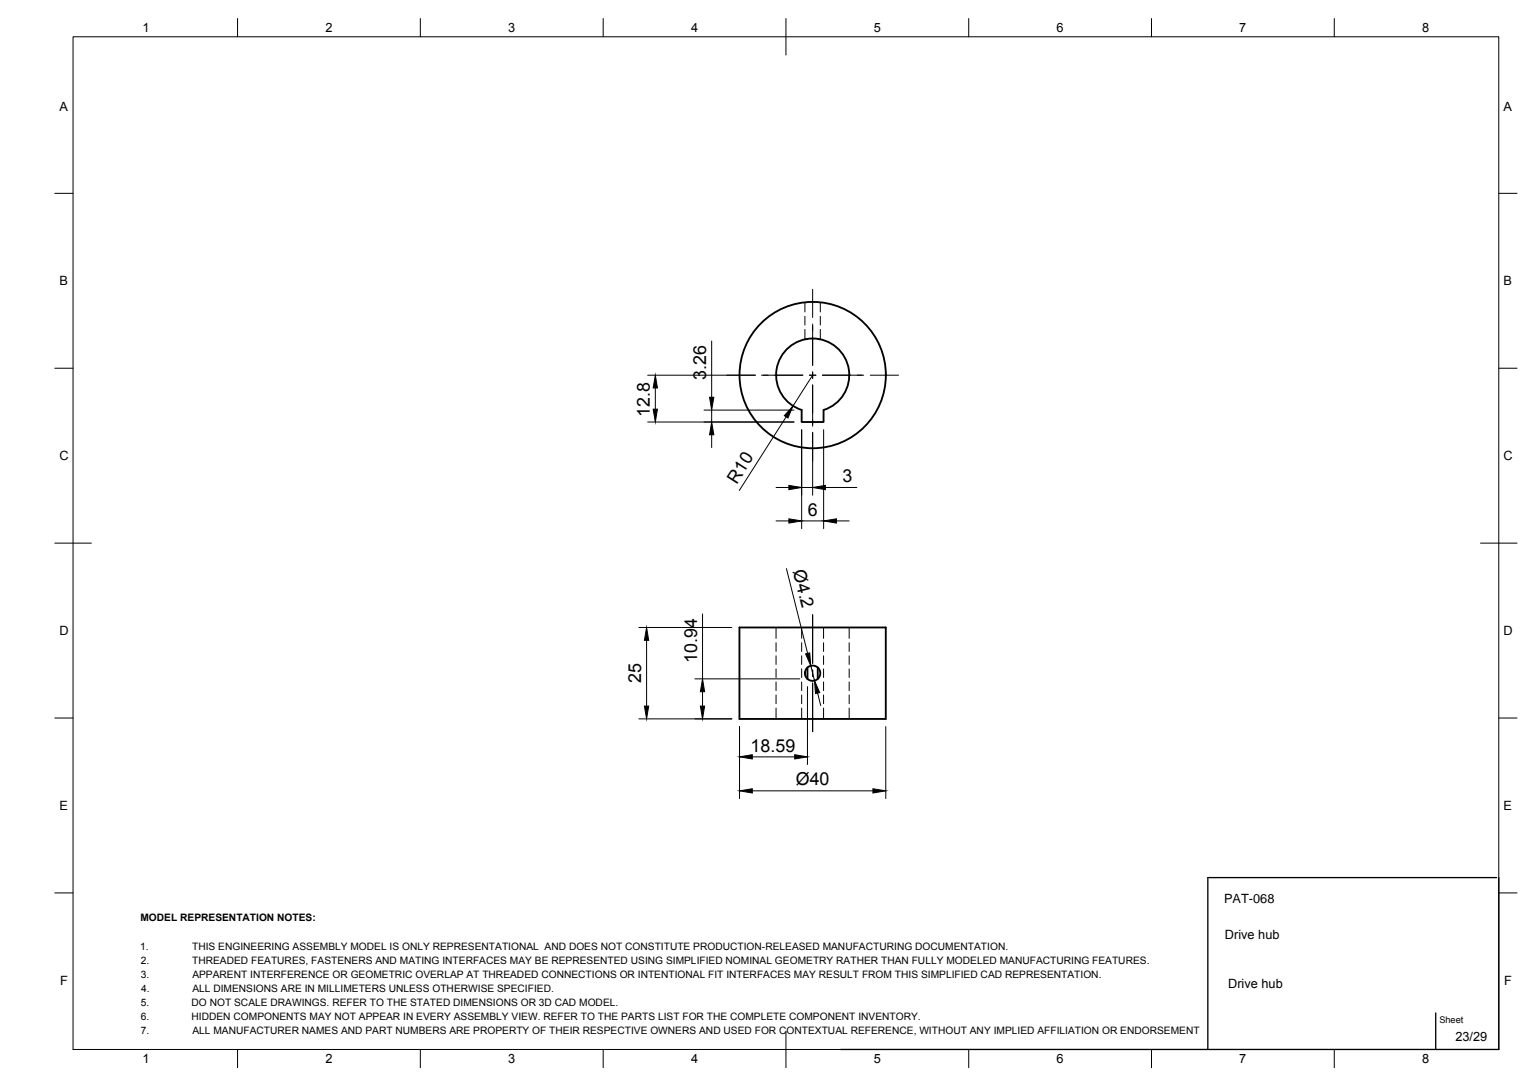
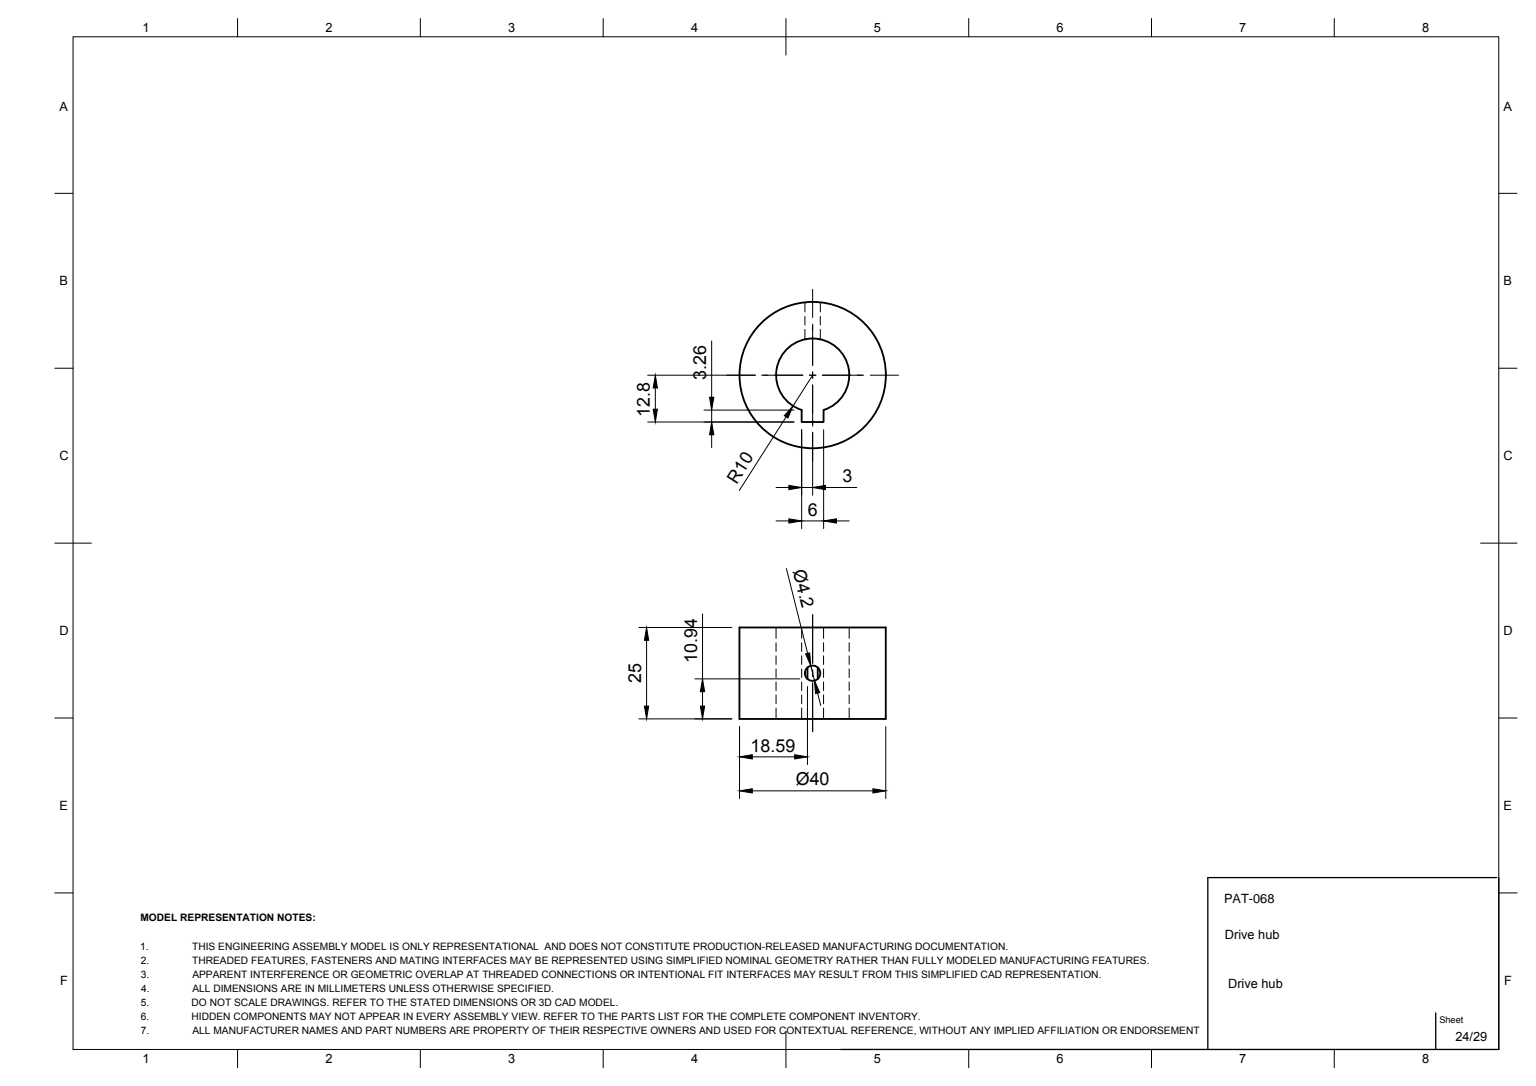
ISO-10303-21;
HEADER;
/* Generated by software containing ST-Developer
 * from STEP Tools, Inc. (www.steptools.com) 
 */

FILE_DESCRIPTION(
/* description */ ('Line shaft on three pillow blocks'),
/* implementation_level */ '2;1');

FILE_NAME(
/* name */ 'Drive hub.step',
/* time_stamp */ '2026-10-27T10:49:19-07:00',
/* author */ (''),
/* organization */ (''),
/* preprocessor_version */ 'ST-DEVELOPER v20.2',
/* originating_system */ 'Autodesk Translation Framework v15.17.0.0',
/* authorisation */ '');

FILE_SCHEMA (('AUTOMOTIVE_DESIGN { 1 0 10303 214 3 1 1 }'));
ENDSEC;

DATA;
#10=MECHANICAL_DESIGN_GEOMETRIC_PRESENTATION_REPRESENTATION('',(#357),#8377);
#247=B_SPLINE_CURVE_WITH_KNOTS('',3,(#7700,#7701,#7702,#7703,#7704,#7705,
#7706,#7707,#7708,#7709),.UNSPECIFIED.,.F.,.F.,(4,2,2,2,4),(0.803821788694085,
0.87295099185362,0.952307212900969,1.03166343394832,1.10079263710785),
 .UNSPECIFIED.);
#248=B_SPLINE_CURVE_WITH_KNOTS('',3,(#7715,#7716,#7717,#7718,#7719,#7720,
#7721,#7722,#7723,#7724,#7725,#7726,#7727,#7728,#7729,#7730,#7731,#7732),
 .UNSPECIFIED.,.F.,.F.,(4,2,2,2,2,2,2,2,4),(0.,0.0791670250779307,0.158334050155861,
0.237500747381213,0.316667444606564,0.395834141831915,0.475000839057267,
0.554167864135197,0.633334889213128),.UNSPECIFIED.);
#249=B_SPLINE_CURVE_WITH_KNOTS('',3,(#7733,#7734,#7735,#7736,#7737,#7738,
#7739,#7740,#7741,#7742,#7743,#7744,#7745,#7746,#7747,#7748,#7749,#7750),
 .UNSPECIFIED.,.F.,.F.,(4,2,2,2,2,2,2,2,4),(0.633334889213128,0.712501914291059,
0.791668939368989,0.870835636594341,0.950002333819692,1.02916903104504,
1.10833572827039,1.18750275334833,1.26666977842626),.UNSPECIFIED.);
#250=B_SPLINE_CURVE_WITH_KNOTS('',3,(#7753,#7754,#7755,#7756,#7757,#7758,
#7759,#7760,#7761,#7762),.UNSPECIFIED.,.F.,.F.,(4,2,2,2,4),(0.168950313426771,
0.238079516586307,0.317435737633656,0.396791958681006,0.465921161840542),
 .UNSPECIFIED.);
#302=SHAPE_REPRESENTATION_RELATIONSHIP('SRR','None',#8519,#329);
#329=ADVANCED_BREP_SHAPE_REPRESENTATION('',(#383),#8368);
#357=STYLED_ITEM('',(#8704),#383);
#383=MANIFOLD_SOLID_BREP('Body1',#4345);
#466=FACE_BOUND('',#1159,.T.);
#467=FACE_BOUND('',#1161,.T.);
#468=FACE_BOUND('',#1163,.T.);
#469=FACE_BOUND('',#1165,.T.);
#598=PLANE('',#4994);
#599=PLANE('',#4999);
#600=PLANE('',#5000);
#601=PLANE('',#5001);
#602=PLANE('',#5002);
#603=PLANE('',#5003);
#604=PLANE('',#5010);
#825=FACE_OUTER_BOUND('',#1152,.T.);
#826=FACE_OUTER_BOUND('',#1153,.T.);
#827=FACE_OUTER_BOUND('',#1154,.T.);
#828=FACE_OUTER_BOUND('',#1155,.T.);
#829=FACE_OUTER_BOUND('',#1156,.T.);
#830=FACE_OUTER_BOUND('',#1157,.T.);
#831=FACE_OUTER_BOUND('',#1158,.T.);
#832=FACE_OUTER_BOUND('',#1160,.T.);
#833=FACE_OUTER_BOUND('',#1162,.T.);
#834=FACE_OUTER_BOUND('',#1164,.T.);
#1152=EDGE_LOOP('',(#3651,#3652));
#1153=EDGE_LOOP('',(#3653,#3654,#3655,#3656,#3657,#3658,#3659,#3660,#3661));
#1154=EDGE_LOOP('',(#3662,#3663,#3664));
#1155=EDGE_LOOP('',(#3665,#3666,#3667,#3668));
#1156=EDGE_LOOP('',(#3669,#3670,#3671,#3672));
#1157=EDGE_LOOP('',(#3673,#3674,#3675,#3676));
#1158=EDGE_LOOP('',(#3677));
#1159=EDGE_LOOP('',(#3678,#3679,#3680,#3681));
#1160=EDGE_LOOP('',(#3682,#3683,#3684,#3685));
#1161=EDGE_LOOP('',(#3686,#3687,#3688,#3689));
#1162=EDGE_LOOP('',(#3690,#3691,#3692,#3693));
#1163=EDGE_LOOP('',(#3694,#3695));
#1164=EDGE_LOOP('',(#3696));
#1165=EDGE_LOOP('',(#3697,#3698,#3699,#3700));
#1471=LINE('',#7696,#1798);
#1472=LINE('',#7713,#1799);
#1473=LINE('',#7764,#1800);
#1474=LINE('',#7768,#1801);
#1475=LINE('',#7770,#1802);
#1476=LINE('',#7772,#1803);
#1477=LINE('',#7773,#1804);
#1478=LINE('',#7776,#1805);
#1479=LINE('',#7778,#1806);
#1480=LINE('',#7779,#1807);
#1481=LINE('',#7782,#1808);
#1482=LINE('',#7784,#1809);
#1483=LINE('',#7785,#1810);
#1484=LINE('',#7794,#1811);
#1798=VECTOR('',#6048,1.);
#1799=VECTOR('',#6055,0.21);
#1800=VECTOR('',#6060,1.);
#1801=VECTOR('',#6063,1.);
#1802=VECTOR('',#6064,1.);
#1803=VECTOR('',#6065,1.);
#1804=VECTOR('',#6066,1.);
#1805=VECTOR('',#6069,1.);
#1806=VECTOR('',#6070,1.);
#1807=VECTOR('',#6071,1.);
#1808=VECTOR('',#6074,1.);
#1809=VECTOR('',#6075,1.);
#1810=VECTOR('',#6076,1.);
#1811=VECTOR('',#6089,2.);
#2020=CIRCLE('',#4995,0.21);
#2021=CIRCLE('',#4997,0.21);
#2022=CIRCLE('',#4998,0.21);
#2023=CIRCLE('',#5004,2.);
#2024=CIRCLE('',#5005,1.);
#2025=CIRCLE('',#5007,1.);
#2026=CIRCLE('',#5009,2.);
#2307=VERTEX_POINT('',#7694);
#2308=VERTEX_POINT('',#7695);
#2309=VERTEX_POINT('',#7699);
#2310=VERTEX_POINT('',#7710);
#2311=VERTEX_POINT('',#7712);
#2312=VERTEX_POINT('',#7714);
#2313=VERTEX_POINT('',#7751);
#2314=VERTEX_POINT('',#7766);
#2315=VERTEX_POINT('',#7767);
#2316=VERTEX_POINT('',#7769);
#2317=VERTEX_POINT('',#7771);
#2318=VERTEX_POINT('',#7775);
#2319=VERTEX_POINT('',#7777);
#2320=VERTEX_POINT('',#7781);
#2321=VERTEX_POINT('',#7783);
#2322=VERTEX_POINT('',#7787);
#2323=VERTEX_POINT('',#7793);
#2774=EDGE_CURVE('',#2307,#2308,#1471,.T.);
#2775=EDGE_CURVE('',#2307,#2308,#2020,.T.);
#2776=EDGE_CURVE('',#2309,#2307,#247,.T.);
#2777=EDGE_CURVE('',#2310,#2309,#2021,.T.);
#2778=EDGE_CURVE('',#2310,#2311,#1472,.T.);
#2779=EDGE_CURVE('',#2312,#2311,#248,.T.);
#2780=EDGE_CURVE('',#2311,#2312,#249,.T.);
#2781=EDGE_CURVE('',#2313,#2310,#2022,.T.);
#2782=EDGE_CURVE('',#2308,#2313,#250,.T.);
#2783=EDGE_CURVE('',#2313,#2309,#1473,.T.);
#2784=EDGE_CURVE('',#2314,#2315,#1474,.T.);
#2785=EDGE_CURVE('',#2314,#2316,#1475,.T.);
#2786=EDGE_CURVE('',#2317,#2316,#1476,.T.);
#2787=EDGE_CURVE('',#2315,#2317,#1477,.T.);
#2788=EDGE_CURVE('',#2318,#2314,#1478,.T.);
#2789=EDGE_CURVE('',#2318,#2319,#1479,.T.);
#2790=EDGE_CURVE('',#2316,#2319,#1480,.T.);
#2791=EDGE_CURVE('',#2320,#2318,#1481,.T.);
#2792=EDGE_CURVE('',#2321,#2320,#1482,.T.);
#2793=EDGE_CURVE('',#2319,#2321,#1483,.T.);
#2794=EDGE_CURVE('',#2322,#2322,#2023,.T.);
#2795=EDGE_CURVE('',#2321,#2317,#2024,.T.);
#2796=EDGE_CURVE('',#2320,#2315,#2025,.T.);
#2797=EDGE_CURVE('',#2322,#2323,#1484,.T.);
#2798=EDGE_CURVE('',#2323,#2323,#2026,.T.);
#3651=ORIENTED_EDGE('',*,*,#2774,.F.);
#3652=ORIENTED_EDGE('',*,*,#2775,.T.);
#3653=ORIENTED_EDGE('',*,*,#2776,.F.);
#3654=ORIENTED_EDGE('',*,*,#2777,.F.);
#3655=ORIENTED_EDGE('',*,*,#2778,.T.);
#3656=ORIENTED_EDGE('',*,*,#2779,.F.);
#3657=ORIENTED_EDGE('',*,*,#2780,.F.);
#3658=ORIENTED_EDGE('',*,*,#2778,.F.);
#3659=ORIENTED_EDGE('',*,*,#2781,.F.);
#3660=ORIENTED_EDGE('',*,*,#2782,.F.);
#3661=ORIENTED_EDGE('',*,*,#2775,.F.);
#3662=ORIENTED_EDGE('',*,*,#2783,.F.);
#3663=ORIENTED_EDGE('',*,*,#2781,.T.);
#3664=ORIENTED_EDGE('',*,*,#2777,.T.);
#3665=ORIENTED_EDGE('',*,*,#2784,.F.);
#3666=ORIENTED_EDGE('',*,*,#2785,.T.);
#3667=ORIENTED_EDGE('',*,*,#2786,.F.);
#3668=ORIENTED_EDGE('',*,*,#2787,.F.);
#3669=ORIENTED_EDGE('',*,*,#2788,.F.);
#3670=ORIENTED_EDGE('',*,*,#2789,.T.);
#3671=ORIENTED_EDGE('',*,*,#2790,.F.);
#3672=ORIENTED_EDGE('',*,*,#2785,.F.);
#3673=ORIENTED_EDGE('',*,*,#2791,.F.);
#3674=ORIENTED_EDGE('',*,*,#2792,.F.);
#3675=ORIENTED_EDGE('',*,*,#2793,.F.);
#3676=ORIENTED_EDGE('',*,*,#2789,.F.);
#3677=ORIENTED_EDGE('',*,*,#2794,.T.);
#3678=ORIENTED_EDGE('',*,*,#2786,.T.);
#3679=ORIENTED_EDGE('',*,*,#2790,.T.);
#3680=ORIENTED_EDGE('',*,*,#2793,.T.);
#3681=ORIENTED_EDGE('',*,*,#2795,.T.);
#3682=ORIENTED_EDGE('',*,*,#2787,.T.);
#3683=ORIENTED_EDGE('',*,*,#2795,.F.);
#3684=ORIENTED_EDGE('',*,*,#2792,.T.);
#3685=ORIENTED_EDGE('',*,*,#2796,.T.);
#3686=ORIENTED_EDGE('',*,*,#2782,.T.);
#3687=ORIENTED_EDGE('',*,*,#2783,.T.);
#3688=ORIENTED_EDGE('',*,*,#2776,.T.);
#3689=ORIENTED_EDGE('',*,*,#2774,.T.);
#3690=ORIENTED_EDGE('',*,*,#2794,.F.);
#3691=ORIENTED_EDGE('',*,*,#2797,.T.);
#3692=ORIENTED_EDGE('',*,*,#2798,.T.);
#3693=ORIENTED_EDGE('',*,*,#2797,.F.);
#3694=ORIENTED_EDGE('',*,*,#2779,.T.);
#3695=ORIENTED_EDGE('',*,*,#2780,.T.);
#3696=ORIENTED_EDGE('',*,*,#2798,.F.);
#3697=ORIENTED_EDGE('',*,*,#2784,.T.);
#3698=ORIENTED_EDGE('',*,*,#2796,.F.);
#3699=ORIENTED_EDGE('',*,*,#2791,.T.);
#3700=ORIENTED_EDGE('',*,*,#2788,.T.);
#4053=CYLINDRICAL_SURFACE('',#4996,0.21);
#4054=CYLINDRICAL_SURFACE('',#5006,1.);
#4055=CYLINDRICAL_SURFACE('',#5008,2.);
#4243=ADVANCED_FACE('',(#825),#598,.T.);
#4244=ADVANCED_FACE('',(#826),#4053,.F.);
#4245=ADVANCED_FACE('',(#827),#599,.T.);
#4246=ADVANCED_FACE('',(#828),#600,.F.);
#4247=ADVANCED_FACE('',(#829),#601,.F.);
#4248=ADVANCED_FACE('',(#830),#602,.F.);
#4249=ADVANCED_FACE('',(#831,#466),#603,.T.);
#4250=ADVANCED_FACE('',(#832,#467),#4054,.F.);
#4251=ADVANCED_FACE('',(#833,#468),#4055,.T.);
#4252=ADVANCED_FACE('',(#834,#469),#604,.F.);
#4345=CLOSED_SHELL('',(#4243,#4244,#4245,#4246,#4247,#4248,#4249,#4250,
#4251,#4252));
#4993=AXIS2_PLACEMENT_3D('',#7692,#6044,#6045);
#4994=AXIS2_PLACEMENT_3D('',#7693,#6046,#6047);
#4995=AXIS2_PLACEMENT_3D('',#7697,#6049,#6050);
#4996=AXIS2_PLACEMENT_3D('',#7698,#6051,#6052);
#4997=AXIS2_PLACEMENT_3D('',#7711,#6053,#6054);
#4998=AXIS2_PLACEMENT_3D('',#7752,#6056,#6057);
#4999=AXIS2_PLACEMENT_3D('',#7763,#6058,#6059);
#5000=AXIS2_PLACEMENT_3D('',#7765,#6061,#6062);
#5001=AXIS2_PLACEMENT_3D('',#7774,#6067,#6068);
#5002=AXIS2_PLACEMENT_3D('',#7780,#6072,#6073);
#5003=AXIS2_PLACEMENT_3D('',#7786,#6077,#6078);
#5004=AXIS2_PLACEMENT_3D('',#7788,#6079,#6080);
#5005=AXIS2_PLACEMENT_3D('',#7789,#6081,#6082);
#5006=AXIS2_PLACEMENT_3D('',#7790,#6083,#6084);
#5007=AXIS2_PLACEMENT_3D('',#7791,#6085,#6086);
#5008=AXIS2_PLACEMENT_3D('',#7792,#6087,#6088);
#5009=AXIS2_PLACEMENT_3D('',#7795,#6090,#6091);
#5010=AXIS2_PLACEMENT_3D('',#7796,#6092,#6093);
#6044=DIRECTION('axis',(0.,0.,1.));
#6045=DIRECTION('refdir',(1.,0.,0.));
#6046=DIRECTION('center_axis',(0.,0.,1.));
#6047=DIRECTION('ref_axis',(1.,0.,0.));
#6048=DIRECTION('',(0.,1.,0.));
#6049=DIRECTION('center_axis',(0.,0.,1.));
#6050=DIRECTION('ref_axis',(1.,0.,0.));
#6051=DIRECTION('center_axis',(0.,0.,1.));
#6052=DIRECTION('ref_axis',(1.,0.,0.));
#6053=DIRECTION('center_axis',(0.,0.,1.));
#6054=DIRECTION('ref_axis',(1.,0.,0.));
#6055=DIRECTION('',(0.,0.,1.));
#6056=DIRECTION('center_axis',(0.,0.,1.));
#6057=DIRECTION('ref_axis',(1.,0.,0.));
#6058=DIRECTION('center_axis',(0.,0.,1.));
#6059=DIRECTION('ref_axis',(1.,0.,0.));
#6060=DIRECTION('',(0.,-1.,0.));
#6061=DIRECTION('center_axis',(-1.,0.,0.));
#6062=DIRECTION('ref_axis',(0.,0.,1.));
#6063=DIRECTION('',(0.,0.,1.));
#6064=DIRECTION('',(0.,1.,0.));
#6065=DIRECTION('',(0.,0.,-1.));
#6066=DIRECTION('',(0.,1.,0.));
#6067=DIRECTION('center_axis',(0.,0.,-1.));
#6068=DIRECTION('ref_axis',(-1.,0.,0.));
#6069=DIRECTION('',(-1.,0.,0.));
#6070=DIRECTION('',(0.,1.,0.));
#6071=DIRECTION('',(1.,0.,0.));
#6072=DIRECTION('center_axis',(1.,0.,0.));
#6073=DIRECTION('ref_axis',(0.,0.,-1.));
#6074=DIRECTION('',(0.,0.,-1.));
#6075=DIRECTION('',(0.,-1.,0.));
#6076=DIRECTION('',(0.,0.,1.));
#6077=DIRECTION('center_axis',(0.,1.,0.));
#6078=DIRECTION('ref_axis',(1.,0.,0.));
#6079=DIRECTION('center_axis',(0.,1.,0.));
#6080=DIRECTION('ref_axis',(1.,0.,0.));
#6081=DIRECTION('center_axis',(0.,-1.,0.));
#6082=DIRECTION('ref_axis',(1.,0.,0.));
#6083=DIRECTION('center_axis',(0.,1.,0.));
#6084=DIRECTION('ref_axis',(-1.83697019872103E-16,0.,1.));
#6085=DIRECTION('center_axis',(0.,-1.,0.));
#6086=DIRECTION('ref_axis',(1.,0.,0.));
#6087=DIRECTION('center_axis',(0.,1.,0.));
#6088=DIRECTION('ref_axis',(1.,0.,0.));
#6089=DIRECTION('',(0.,-1.,0.));
#6090=DIRECTION('center_axis',(0.,1.,0.));
#6091=DIRECTION('ref_axis',(1.,0.,0.));
#6092=DIRECTION('center_axis',(0.,1.,0.));
#6093=DIRECTION('ref_axis',(1.,0.,0.));
#7692=CARTESIAN_POINT('',(0.,0.,0.));
#7693=CARTESIAN_POINT('Origin',(0.,7.25,5.52));
#7694=CARTESIAN_POINT('',(0.141067359796651,7.09443650813895,5.52));
#7695=CARTESIAN_POINT('',(0.141067359796651,7.40556349186105,5.52));
#7696=CARTESIAN_POINT('',(0.141067359796651,6.,5.52));
#7697=CARTESIAN_POINT('Origin',(0.,7.25,5.52));
#7698=CARTESIAN_POINT('Origin',(0.,7.25,5.52));
#7699=CARTESIAN_POINT('',(-0.141067359796651,7.09443650813895,5.52));
#7700=CARTESIAN_POINT('Ctrl Pts',(-0.141067359796651,7.09443650813895,5.52));
#7701=CARTESIAN_POINT('Ctrl Pts',(-0.12381835669822,7.0787948476368,5.52245784982447));
#7702=CARTESIAN_POINT('Ctrl Pts',(-0.102998643109696,7.06537595666898,5.52493819304946));
#7703=CARTESIAN_POINT('Ctrl Pts',(-0.0546141143983527,7.04530253627557,
5.52884449237241));
#7704=CARTESIAN_POINT('Ctrl Pts',(-0.0264520736824499,7.04,5.53));
#7705=CARTESIAN_POINT('Ctrl Pts',(0.0264520736824498,7.04,5.53));
#7706=CARTESIAN_POINT('Ctrl Pts',(0.0546141143983529,7.04530253627557,5.52884449237241));
#7707=CARTESIAN_POINT('Ctrl Pts',(0.102998643109696,7.06537595666898,5.52493819304946));
#7708=CARTESIAN_POINT('Ctrl Pts',(0.123818356698219,7.0787948476368,5.52245784982447));
#7709=CARTESIAN_POINT('Ctrl Pts',(0.141067359796651,7.09443650813895,5.52));
#7710=CARTESIAN_POINT('',(-0.21,7.25,5.52));
#7711=CARTESIAN_POINT('Origin',(0.,7.25,5.52));
#7712=CARTESIAN_POINT('',(-0.21,7.25,6.51894444366855));
#7713=CARTESIAN_POINT('',(-0.21,7.25,5.52));
#7714=CARTESIAN_POINT('',(0.21,7.25,6.51894444366855));
#7715=CARTESIAN_POINT('Ctrl Pts',(0.21,7.25,6.51894444366855));
#7716=CARTESIAN_POINT('Ctrl Pts',(0.21,7.22361099164069,6.51894444366855));
#7717=CARTESIAN_POINT('Ctrl Pts',(0.204722164681422,7.19547640622183,6.51952376620524));
#7718=CARTESIAN_POINT('Ctrl Pts',(0.183284867450471,7.14374255317885,6.52161307432363));
#7719=CARTESIAN_POINT('Ctrl Pts',(0.167126466290584,7.12014161819223,6.52309254589373));
#7720=CARTESIAN_POINT('Ctrl Pts',(0.129858458976497,7.08287361087815,6.52586721250997));
#7721=CARTESIAN_POINT('Ctrl Pts',(0.106257490219277,7.06671514943451,6.527343117591));
#7722=CARTESIAN_POINT('Ctrl Pts',(0.054523523784787,7.04527780741314,6.52942425936951));
#7723=CARTESIAN_POINT('Ctrl Pts',(0.0263888990751171,7.04,6.53));
#7724=CARTESIAN_POINT('Ctrl Pts',(-0.0263888990751171,7.04,6.53));
#7725=CARTESIAN_POINT('Ctrl Pts',(-0.0545235237847869,7.04527780741314,
6.52942425936951));
#7726=CARTESIAN_POINT('Ctrl Pts',(-0.106257490219277,7.06671514943451,6.527343117591));
#7727=CARTESIAN_POINT('Ctrl Pts',(-0.129858458976497,7.08287361087815,6.52586721250997));
#7728=CARTESIAN_POINT('Ctrl Pts',(-0.167126466290584,7.12014161819223,6.52309254589373));
#7729=CARTESIAN_POINT('Ctrl Pts',(-0.183284867450471,7.14374255317885,6.52161307432363));
#7730=CARTESIAN_POINT('Ctrl Pts',(-0.204722164681422,7.19547640622183,6.51952376620524));
#7731=CARTESIAN_POINT('Ctrl Pts',(-0.21,7.22361099164069,6.51894444366855));
#7732=CARTESIAN_POINT('Ctrl Pts',(-0.21,7.25,6.51894444366855));
#7733=CARTESIAN_POINT('Ctrl Pts',(-0.21,7.25,6.51894444366855));
#7734=CARTESIAN_POINT('Ctrl Pts',(-0.21,7.27638900835931,6.51894444366855));
#7735=CARTESIAN_POINT('Ctrl Pts',(-0.204722164681422,7.30452359377817,6.51952376620524));
#7736=CARTESIAN_POINT('Ctrl Pts',(-0.183284867450471,7.35625744682115,6.52161307432363));
#7737=CARTESIAN_POINT('Ctrl Pts',(-0.167126466290584,7.37985838180777,6.52309254589373));
#7738=CARTESIAN_POINT('Ctrl Pts',(-0.129858458976497,7.41712638912185,6.52586721250997));
#7739=CARTESIAN_POINT('Ctrl Pts',(-0.106257490219277,7.43328485056549,6.527343117591));
#7740=CARTESIAN_POINT('Ctrl Pts',(-0.054523523784787,7.45472219258686,6.52942425936951));
#7741=CARTESIAN_POINT('Ctrl Pts',(-0.0263888990751171,7.46,6.53));
#7742=CARTESIAN_POINT('Ctrl Pts',(0.026388899075117,7.46,6.53));
#7743=CARTESIAN_POINT('Ctrl Pts',(0.0545235237847869,7.45472219258686,6.52942425936951));
#7744=CARTESIAN_POINT('Ctrl Pts',(0.106257490219278,7.43328485056549,6.527343117591));
#7745=CARTESIAN_POINT('Ctrl Pts',(0.129858458976496,7.41712638912185,6.52586721250997));
#7746=CARTESIAN_POINT('Ctrl Pts',(0.167126466290584,7.37985838180777,6.52309254589373));
#7747=CARTESIAN_POINT('Ctrl Pts',(0.183284867450471,7.35625744682115,6.52161307432363));
#7748=CARTESIAN_POINT('Ctrl Pts',(0.204722164681422,7.30452359377817,6.51952376620524));
#7749=CARTESIAN_POINT('Ctrl Pts',(0.21,7.27638900835931,6.51894444366855));
#7750=CARTESIAN_POINT('Ctrl Pts',(0.21,7.25,6.51894444366855));
#7751=CARTESIAN_POINT('',(-0.141067359796651,7.40556349186105,5.52));
#7752=CARTESIAN_POINT('Origin',(0.,7.25,5.52));
#7753=CARTESIAN_POINT('Ctrl Pts',(0.141067359796651,7.40556349186105,5.52));
#7754=CARTESIAN_POINT('Ctrl Pts',(0.123818356698219,7.4212051523632,5.52245784982447));
#7755=CARTESIAN_POINT('Ctrl Pts',(0.102998643109696,7.43462404333102,5.52493819304946));
#7756=CARTESIAN_POINT('Ctrl Pts',(0.0546141143983527,7.45469746372443,5.52884449237241));
#7757=CARTESIAN_POINT('Ctrl Pts',(0.0264520736824498,7.46,5.53));
#7758=CARTESIAN_POINT('Ctrl Pts',(-0.0264520736824498,7.46,5.53));
#7759=CARTESIAN_POINT('Ctrl Pts',(-0.0546141143983527,7.45469746372443,
5.52884449237241));
#7760=CARTESIAN_POINT('Ctrl Pts',(-0.102998643109696,7.43462404333102,5.52493819304946));
#7761=CARTESIAN_POINT('Ctrl Pts',(-0.123818356698219,7.4212051523632,5.52245784982447));
#7762=CARTESIAN_POINT('Ctrl Pts',(-0.141067359796651,7.40556349186105,5.52));
#7763=CARTESIAN_POINT('Origin',(0.,7.25,5.52));
#7764=CARTESIAN_POINT('',(-0.141067359796651,6.,5.52));
#7765=CARTESIAN_POINT('Origin',(-0.3,5.9,3.25));
#7766=CARTESIAN_POINT('',(-0.3,6.,3.25));
#7767=CARTESIAN_POINT('',(-0.3,6.,3.57606079858305));
#7768=CARTESIAN_POINT('',(-0.3,6.,3.89));
#7769=CARTESIAN_POINT('',(-0.3,8.5,3.25));
#7770=CARTESIAN_POINT('',(-0.3,5.9,3.25));
#7771=CARTESIAN_POINT('',(-0.3,8.5,3.57606079858305));
#7772=CARTESIAN_POINT('',(-0.3,8.5,3.89));
#7773=CARTESIAN_POINT('',(-0.3,6.,3.57606079858305));
#7774=CARTESIAN_POINT('Origin',(0.3,5.9,3.25));
#7775=CARTESIAN_POINT('',(0.3,6.,3.25));
#7776=CARTESIAN_POINT('',(0.15,6.,3.25));
#7777=CARTESIAN_POINT('',(0.3,8.5,3.25));
#7778=CARTESIAN_POINT('',(0.3,5.9,3.25));
#7779=CARTESIAN_POINT('',(0.15,8.5,3.25));
#7780=CARTESIAN_POINT('Origin',(0.3,5.9,4.53));
#7781=CARTESIAN_POINT('',(0.3,6.,3.57606079858305));
#7782=CARTESIAN_POINT('',(0.3,6.,4.53));
#7783=CARTESIAN_POINT('',(0.3,8.5,3.57606079858305));
#7784=CARTESIAN_POINT('',(0.3,6.,3.57606079858305));
#7785=CARTESIAN_POINT('',(0.3,8.5,4.53));
#7786=CARTESIAN_POINT('Origin',(0.,8.5,4.53));
#7787=CARTESIAN_POINT('',(-2.,8.5,4.53));
#7788=CARTESIAN_POINT('Origin',(0.,8.5,4.53));
#7789=CARTESIAN_POINT('Origin',(0.,8.5,4.53));
#7790=CARTESIAN_POINT('Origin',(0.,6.,4.53));
#7791=CARTESIAN_POINT('Origin',(0.,6.,4.53));
#7792=CARTESIAN_POINT('Origin',(0.,6.,4.53));
#7793=CARTESIAN_POINT('',(-2.,6.,4.53));
#7794=CARTESIAN_POINT('',(-2.,6.,4.53));
#7795=CARTESIAN_POINT('Origin',(0.,6.,4.53));
#7796=CARTESIAN_POINT('Origin',(0.,6.,4.53));
#8336=UNCERTAINTY_MEASURE_WITH_UNIT(LENGTH_MEASURE(0.001),#8378,
'DISTANCE_ACCURACY_VALUE',
'Maximum model space distance between geometric entities at asserted c
onnectivities');
#8345=UNCERTAINTY_MEASURE_WITH_UNIT(LENGTH_MEASURE(0.001),#8378,
'DISTANCE_ACCURACY_VALUE',
'Maximum model space distance between geometric entities at asserted c
onnectivities');
#8368=(
GEOMETRIC_REPRESENTATION_CONTEXT(3)
GLOBAL_UNCERTAINTY_ASSIGNED_CONTEXT((#8336))
GLOBAL_UNIT_ASSIGNED_CONTEXT((#8378,#8380,#8381))
REPRESENTATION_CONTEXT('','3D')
);
#8377=(
GEOMETRIC_REPRESENTATION_CONTEXT(3)
GLOBAL_UNCERTAINTY_ASSIGNED_CONTEXT((#8345))
GLOBAL_UNIT_ASSIGNED_CONTEXT((#8378,#8380,#8381))
REPRESENTATION_CONTEXT('','3D')
);
#8378=(
LENGTH_UNIT()
NAMED_UNIT(*)
SI_UNIT(.CENTI.,.METRE.)
);
#8380=(
NAMED_UNIT(*)
PLANE_ANGLE_UNIT()
SI_UNIT($,.RADIAN.)
);
#8381=(
NAMED_UNIT(*)
SI_UNIT($,.STERADIAN.)
SOLID_ANGLE_UNIT()
);
#8404=SHAPE_DEFINITION_REPRESENTATION(#8471,#8519);
#8471=PRODUCT_DEFINITION_SHAPE('',$,#8551);
#8519=SHAPE_REPRESENTATION('',(#4993),#8368);
#8528=PRODUCT_DEFINITION_CONTEXT('part definition',#8623,'design');
#8551=PRODUCT_DEFINITION('Drive hub','Drive hub',#8582,#8528);
#8582=PRODUCT_DEFINITION_FORMATION('',$,#8647);
#8623=APPLICATION_CONTEXT(
'Core Data for Automotive Mechanical Design Process');
#8624=PRODUCT_CONTEXT('part definition',#8623,'mechanical');
#8647=PRODUCT('Drive hub','Drive hub','Drive hub',(#8624));
#8698=COLOUR_RGB('Light Blue',0.38,0.62,0.78);
#8699=FILL_AREA_STYLE_COLOUR('',#8698);
#8700=FILL_AREA_STYLE('',(#8699));
#8701=SURFACE_STYLE_FILL_AREA(#8700);
#8702=SURFACE_SIDE_STYLE('',(#8701));
#8703=SURFACE_STYLE_USAGE(.BOTH.,#8702);
#8704=PRESENTATION_STYLE_ASSIGNMENT((#8703));
ENDSEC;
END-ISO-10303-21;
